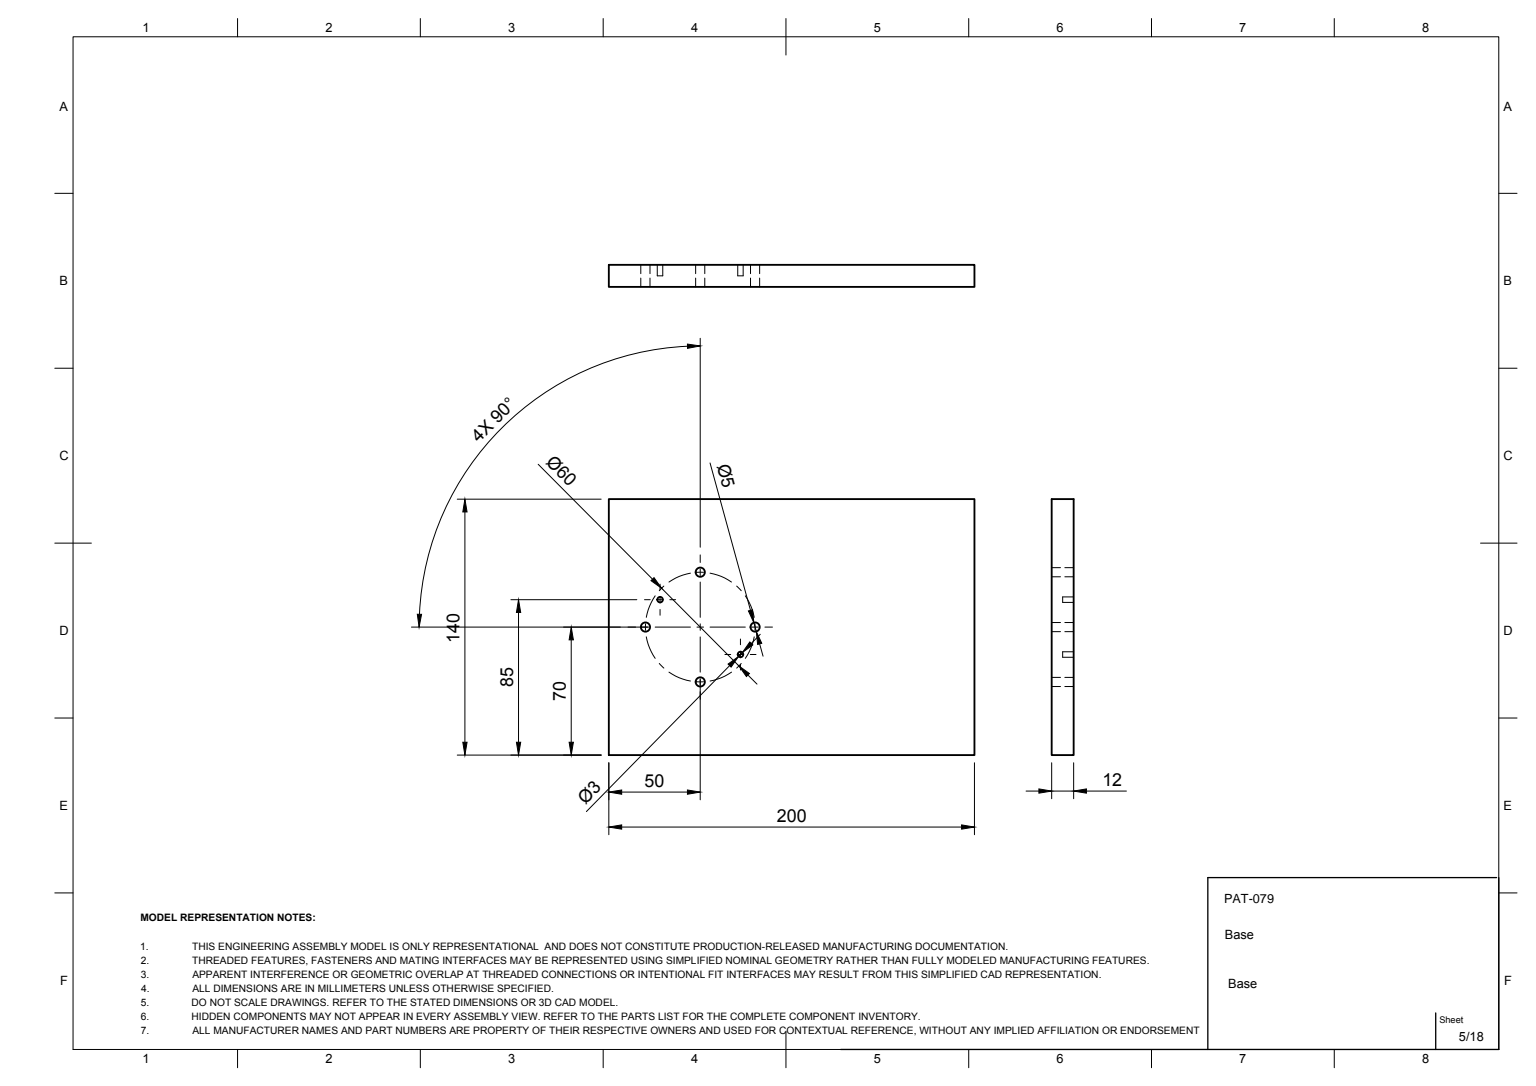
ISO-10303-21;
HEADER;
/* Generated by software containing ST-Developer
 * from STEP Tools, Inc. (www.steptools.com) 
 */

FILE_DESCRIPTION(
/* description */ ('Pipe clamp stand with threaded column'),
/* implementation_level */ '2;1');

FILE_NAME(
/* name */ 'Base.step',
/* time_stamp */ '2026-10-27T10:55:48-07:00',
/* author */ (''),
/* organization */ (''),
/* preprocessor_version */ 'ST-DEVELOPER v20.2',
/* originating_system */ 'Autodesk Translation Framework v15.17.0.0',
/* authorisation */ '');

FILE_SCHEMA (('AUTOMOTIVE_DESIGN { 1 0 10303 214 3 1 1 }'));
ENDSEC;

DATA;
#10=MECHANICAL_DESIGN_GEOMETRIC_PRESENTATION_REPRESENTATION('',(#741),#34433);
#697=SHAPE_REPRESENTATION_RELATIONSHIP('SRR','None',#34539,#719);
#719=ADVANCED_BREP_SHAPE_REPRESENTATION('',(#771),#34407);
#741=STYLED_ITEM('',(#34722),#771);
#771=MANIFOLD_SOLID_BREP('Body1',#8768);
#799=FACE_BOUND('',#1544,.T.);
#800=FACE_BOUND('',#1545,.T.);
#801=FACE_BOUND('',#1546,.T.);
#802=FACE_BOUND('',#1547,.T.);
#803=FACE_BOUND('',#1548,.T.);
#804=FACE_BOUND('',#1549,.T.);
#805=FACE_BOUND('',#1551,.T.);
#806=FACE_BOUND('',#1552,.T.);
#807=FACE_BOUND('',#1553,.T.);
#808=FACE_BOUND('',#1554,.T.);
#857=PLANE('',#9049);
#858=PLANE('',#9053);
#859=PLANE('',#9066);
#860=PLANE('',#9067);
#861=PLANE('',#9068);
#862=PLANE('',#9069);
#863=PLANE('',#9070);
#864=PLANE('',#9071);
#1044=FACE_OUTER_BOUND('',#1531,.T.);
#1045=FACE_OUTER_BOUND('',#1532,.T.);
#1046=FACE_OUTER_BOUND('',#1533,.T.);
#1047=FACE_OUTER_BOUND('',#1534,.T.);
#1048=FACE_OUTER_BOUND('',#1535,.T.);
#1049=FACE_OUTER_BOUND('',#1536,.T.);
#1050=FACE_OUTER_BOUND('',#1537,.T.);
#1051=FACE_OUTER_BOUND('',#1538,.T.);
#1052=FACE_OUTER_BOUND('',#1539,.T.);
#1053=FACE_OUTER_BOUND('',#1540,.T.);
#1054=FACE_OUTER_BOUND('',#1541,.T.);
#1055=FACE_OUTER_BOUND('',#1542,.T.);
#1056=FACE_OUTER_BOUND('',#1543,.T.);
#1057=FACE_OUTER_BOUND('',#1550,.T.);
#1531=EDGE_LOOP('',(#5513,#5514,#5515,#5516));
#1532=EDGE_LOOP('',(#5517));
#1533=EDGE_LOOP('',(#5518,#5519,#5520,#5521));
#1534=EDGE_LOOP('',(#5522));
#1535=EDGE_LOOP('',(#5523,#5524,#5525,#5526));
#1536=EDGE_LOOP('',(#5527,#5528,#5529,#5530));
#1537=EDGE_LOOP('',(#5531,#5532,#5533,#5534));
#1538=EDGE_LOOP('',(#5535,#5536,#5537,#5538));
#1539=EDGE_LOOP('',(#5539,#5540,#5541,#5542));
#1540=EDGE_LOOP('',(#5543,#5544,#5545,#5546));
#1541=EDGE_LOOP('',(#5547,#5548,#5549,#5550));
#1542=EDGE_LOOP('',(#5551,#5552,#5553,#5554));
#1543=EDGE_LOOP('',(#5555,#5556,#5557,#5558));
#1544=EDGE_LOOP('',(#5559));
#1545=EDGE_LOOP('',(#5560));
#1546=EDGE_LOOP('',(#5561));
#1547=EDGE_LOOP('',(#5562));
#1548=EDGE_LOOP('',(#5563));
#1549=EDGE_LOOP('',(#5564));
#1550=EDGE_LOOP('',(#5565,#5566,#5567,#5568));
#1551=EDGE_LOOP('',(#5569));
#1552=EDGE_LOOP('',(#5570));
#1553=EDGE_LOOP('',(#5571));
#1554=EDGE_LOOP('',(#5572));
#2076=LINE('',#11713,#2693);
#2077=LINE('',#11720,#2694);
#2078=LINE('',#11727,#2695);
#2079=LINE('',#11733,#2696);
#2080=LINE('',#11739,#2697);
#2081=LINE('',#11745,#2698);
#2082=LINE('',#11750,#2699);
#2083=LINE('',#11752,#2700);
#2084=LINE('',#11754,#2701);
#2085=LINE('',#11755,#2702);
#2086=LINE('',#11758,#2703);
#2087=LINE('',#11760,#2704);
#2088=LINE('',#11761,#2705);
#2089=LINE('',#11764,#2706);
#2090=LINE('',#11766,#2707);
#2091=LINE('',#11767,#2708);
#2092=LINE('',#11769,#2709);
#2093=LINE('',#11770,#2710);
#2693=VECTOR('',#9735,0.15);
#2694=VECTOR('',#9744,0.15);
#2695=VECTOR('',#9753,0.25);
#2696=VECTOR('',#9760,0.25);
#2697=VECTOR('',#9767,0.25);
#2698=VECTOR('',#9774,0.25);
#2699=VECTOR('',#9779,1.);
#2700=VECTOR('',#9780,1.);
#2701=VECTOR('',#9781,1.);
#2702=VECTOR('',#9782,1.);
#2703=VECTOR('',#9785,1.);
#2704=VECTOR('',#9786,1.);
#2705=VECTOR('',#9787,1.);
#2706=VECTOR('',#9790,1.);
#2707=VECTOR('',#9791,1.);
#2708=VECTOR('',#9792,1.);
#2709=VECTOR('',#9795,1.);
#2710=VECTOR('',#9796,1.);
#3310=CIRCLE('',#9047,0.15);
#3311=CIRCLE('',#9048,0.15);
#3312=CIRCLE('',#9051,0.15);
#3313=CIRCLE('',#9052,0.15);
#3314=CIRCLE('',#9055,0.25);
#3315=CIRCLE('',#9056,0.25);
#3316=CIRCLE('',#9058,0.25);
#3317=CIRCLE('',#9059,0.25);
#3318=CIRCLE('',#9061,0.25);
#3319=CIRCLE('',#9062,0.25);
#3320=CIRCLE('',#9064,0.25);
#3321=CIRCLE('',#9065,0.25);
#3444=VERTEX_POINT('',#11710);
#3445=VERTEX_POINT('',#11712);
#3446=VERTEX_POINT('',#11717);
#3447=VERTEX_POINT('',#11719);
#3448=VERTEX_POINT('',#11724);
#3449=VERTEX_POINT('',#11726);
#3450=VERTEX_POINT('',#11730);
#3451=VERTEX_POINT('',#11732);
#3452=VERTEX_POINT('',#11736);
#3453=VERTEX_POINT('',#11738);
#3454=VERTEX_POINT('',#11742);
#3455=VERTEX_POINT('',#11744);
#3456=VERTEX_POINT('',#11748);
#3457=VERTEX_POINT('',#11749);
#3458=VERTEX_POINT('',#11751);
#3459=VERTEX_POINT('',#11753);
#3460=VERTEX_POINT('',#11757);
#3461=VERTEX_POINT('',#11759);
#3462=VERTEX_POINT('',#11763);
#3463=VERTEX_POINT('',#11765);
#4270=EDGE_CURVE('',#3444,#3444,#3310,.T.);
#4271=EDGE_CURVE('',#3444,#3445,#2076,.T.);
#4272=EDGE_CURVE('',#3445,#3445,#3311,.T.);
#4273=EDGE_CURVE('',#3446,#3446,#3312,.T.);
#4274=EDGE_CURVE('',#3446,#3447,#2077,.T.);
#4275=EDGE_CURVE('',#3447,#3447,#3313,.T.);
#4276=EDGE_CURVE('',#3448,#3448,#3314,.T.);
#4277=EDGE_CURVE('',#3448,#3449,#2078,.T.);
#4278=EDGE_CURVE('',#3449,#3449,#3315,.T.);
#4279=EDGE_CURVE('',#3450,#3450,#3316,.T.);
#4280=EDGE_CURVE('',#3450,#3451,#2079,.T.);
#4281=EDGE_CURVE('',#3451,#3451,#3317,.T.);
#4282=EDGE_CURVE('',#3452,#3452,#3318,.T.);
#4283=EDGE_CURVE('',#3452,#3453,#2080,.T.);
#4284=EDGE_CURVE('',#3453,#3453,#3319,.T.);
#4285=EDGE_CURVE('',#3454,#3454,#3320,.T.);
#4286=EDGE_CURVE('',#3454,#3455,#2081,.T.);
#4287=EDGE_CURVE('',#3455,#3455,#3321,.T.);
#4288=EDGE_CURVE('',#3456,#3457,#2082,.T.);
#4289=EDGE_CURVE('',#3457,#3458,#2083,.T.);
#4290=EDGE_CURVE('',#3459,#3458,#2084,.T.);
#4291=EDGE_CURVE('',#3456,#3459,#2085,.T.);
#4292=EDGE_CURVE('',#3460,#3456,#2086,.T.);
#4293=EDGE_CURVE('',#3461,#3459,#2087,.T.);
#4294=EDGE_CURVE('',#3460,#3461,#2088,.T.);
#4295=EDGE_CURVE('',#3462,#3460,#2089,.T.);
#4296=EDGE_CURVE('',#3463,#3461,#2090,.T.);
#4297=EDGE_CURVE('',#3462,#3463,#2091,.T.);
#4298=EDGE_CURVE('',#3457,#3462,#2092,.T.);
#4299=EDGE_CURVE('',#3458,#3463,#2093,.T.);
#5513=ORIENTED_EDGE('',*,*,#4270,.F.);
#5514=ORIENTED_EDGE('',*,*,#4271,.T.);
#5515=ORIENTED_EDGE('',*,*,#4272,.F.);
#5516=ORIENTED_EDGE('',*,*,#4271,.F.);
#5517=ORIENTED_EDGE('',*,*,#4270,.T.);
#5518=ORIENTED_EDGE('',*,*,#4273,.F.);
#5519=ORIENTED_EDGE('',*,*,#4274,.T.);
#5520=ORIENTED_EDGE('',*,*,#4275,.F.);
#5521=ORIENTED_EDGE('',*,*,#4274,.F.);
#5522=ORIENTED_EDGE('',*,*,#4273,.T.);
#5523=ORIENTED_EDGE('',*,*,#4276,.F.);
#5524=ORIENTED_EDGE('',*,*,#4277,.T.);
#5525=ORIENTED_EDGE('',*,*,#4278,.F.);
#5526=ORIENTED_EDGE('',*,*,#4277,.F.);
#5527=ORIENTED_EDGE('',*,*,#4279,.F.);
#5528=ORIENTED_EDGE('',*,*,#4280,.T.);
#5529=ORIENTED_EDGE('',*,*,#4281,.F.);
#5530=ORIENTED_EDGE('',*,*,#4280,.F.);
#5531=ORIENTED_EDGE('',*,*,#4282,.F.);
#5532=ORIENTED_EDGE('',*,*,#4283,.T.);
#5533=ORIENTED_EDGE('',*,*,#4284,.F.);
#5534=ORIENTED_EDGE('',*,*,#4283,.F.);
#5535=ORIENTED_EDGE('',*,*,#4285,.F.);
#5536=ORIENTED_EDGE('',*,*,#4286,.T.);
#5537=ORIENTED_EDGE('',*,*,#4287,.F.);
#5538=ORIENTED_EDGE('',*,*,#4286,.F.);
#5539=ORIENTED_EDGE('',*,*,#4288,.T.);
#5540=ORIENTED_EDGE('',*,*,#4289,.T.);
#5541=ORIENTED_EDGE('',*,*,#4290,.F.);
#5542=ORIENTED_EDGE('',*,*,#4291,.F.);
#5543=ORIENTED_EDGE('',*,*,#4292,.T.);
#5544=ORIENTED_EDGE('',*,*,#4291,.T.);
#5545=ORIENTED_EDGE('',*,*,#4293,.F.);
#5546=ORIENTED_EDGE('',*,*,#4294,.F.);
#5547=ORIENTED_EDGE('',*,*,#4295,.T.);
#5548=ORIENTED_EDGE('',*,*,#4294,.T.);
#5549=ORIENTED_EDGE('',*,*,#4296,.F.);
#5550=ORIENTED_EDGE('',*,*,#4297,.F.);
#5551=ORIENTED_EDGE('',*,*,#4298,.T.);
#5552=ORIENTED_EDGE('',*,*,#4297,.T.);
#5553=ORIENTED_EDGE('',*,*,#4299,.F.);
#5554=ORIENTED_EDGE('',*,*,#4289,.F.);
#5555=ORIENTED_EDGE('',*,*,#4299,.T.);
#5556=ORIENTED_EDGE('',*,*,#4296,.T.);
#5557=ORIENTED_EDGE('',*,*,#4293,.T.);
#5558=ORIENTED_EDGE('',*,*,#4290,.T.);
#5559=ORIENTED_EDGE('',*,*,#4272,.T.);
#5560=ORIENTED_EDGE('',*,*,#4275,.T.);
#5561=ORIENTED_EDGE('',*,*,#4278,.T.);
#5562=ORIENTED_EDGE('',*,*,#4281,.T.);
#5563=ORIENTED_EDGE('',*,*,#4284,.T.);
#5564=ORIENTED_EDGE('',*,*,#4287,.T.);
#5565=ORIENTED_EDGE('',*,*,#4298,.F.);
#5566=ORIENTED_EDGE('',*,*,#4288,.F.);
#5567=ORIENTED_EDGE('',*,*,#4292,.F.);
#5568=ORIENTED_EDGE('',*,*,#4295,.F.);
#5569=ORIENTED_EDGE('',*,*,#4276,.T.);
#5570=ORIENTED_EDGE('',*,*,#4279,.T.);
#5571=ORIENTED_EDGE('',*,*,#4282,.T.);
#5572=ORIENTED_EDGE('',*,*,#4285,.T.);
#7999=CYLINDRICAL_SURFACE('',#9046,0.15);
#8000=CYLINDRICAL_SURFACE('',#9050,0.15);
#8001=CYLINDRICAL_SURFACE('',#9054,0.25);
#8002=CYLINDRICAL_SURFACE('',#9057,0.25);
#8003=CYLINDRICAL_SURFACE('',#9060,0.25);
#8004=CYLINDRICAL_SURFACE('',#9063,0.25);
#8281=ADVANCED_FACE('',(#1044),#7999,.F.);
#8282=ADVANCED_FACE('',(#1045),#857,.T.);
#8283=ADVANCED_FACE('',(#1046),#8000,.F.);
#8284=ADVANCED_FACE('',(#1047),#858,.T.);
#8285=ADVANCED_FACE('',(#1048),#8001,.F.);
#8286=ADVANCED_FACE('',(#1049),#8002,.F.);
#8287=ADVANCED_FACE('',(#1050),#8003,.F.);
#8288=ADVANCED_FACE('',(#1051),#8004,.F.);
#8289=ADVANCED_FACE('',(#1052),#859,.T.);
#8290=ADVANCED_FACE('',(#1053),#860,.T.);
#8291=ADVANCED_FACE('',(#1054),#861,.T.);
#8292=ADVANCED_FACE('',(#1055),#862,.T.);
#8293=ADVANCED_FACE('',(#1056,#799,#800,#801,#802,#803,#804),#863,.T.);
#8294=ADVANCED_FACE('',(#1057,#805,#806,#807,#808),#864,.F.);
#8768=CLOSED_SHELL('',(#8281,#8282,#8283,#8284,#8285,#8286,#8287,#8288,
#8289,#8290,#8291,#8292,#8293,#8294));
#9045=AXIS2_PLACEMENT_3D('',#11708,#9729,#9730);
#9046=AXIS2_PLACEMENT_3D('',#11709,#9731,#9732);
#9047=AXIS2_PLACEMENT_3D('',#11711,#9733,#9734);
#9048=AXIS2_PLACEMENT_3D('',#11714,#9736,#9737);
#9049=AXIS2_PLACEMENT_3D('',#11715,#9738,#9739);
#9050=AXIS2_PLACEMENT_3D('',#11716,#9740,#9741);
#9051=AXIS2_PLACEMENT_3D('',#11718,#9742,#9743);
#9052=AXIS2_PLACEMENT_3D('',#11721,#9745,#9746);
#9053=AXIS2_PLACEMENT_3D('',#11722,#9747,#9748);
#9054=AXIS2_PLACEMENT_3D('',#11723,#9749,#9750);
#9055=AXIS2_PLACEMENT_3D('',#11725,#9751,#9752);
#9056=AXIS2_PLACEMENT_3D('',#11728,#9754,#9755);
#9057=AXIS2_PLACEMENT_3D('',#11729,#9756,#9757);
#9058=AXIS2_PLACEMENT_3D('',#11731,#9758,#9759);
#9059=AXIS2_PLACEMENT_3D('',#11734,#9761,#9762);
#9060=AXIS2_PLACEMENT_3D('',#11735,#9763,#9764);
#9061=AXIS2_PLACEMENT_3D('',#11737,#9765,#9766);
#9062=AXIS2_PLACEMENT_3D('',#11740,#9768,#9769);
#9063=AXIS2_PLACEMENT_3D('',#11741,#9770,#9771);
#9064=AXIS2_PLACEMENT_3D('',#11743,#9772,#9773);
#9065=AXIS2_PLACEMENT_3D('',#11746,#9775,#9776);
#9066=AXIS2_PLACEMENT_3D('',#11747,#9777,#9778);
#9067=AXIS2_PLACEMENT_3D('',#11756,#9783,#9784);
#9068=AXIS2_PLACEMENT_3D('',#11762,#9788,#9789);
#9069=AXIS2_PLACEMENT_3D('',#11768,#9793,#9794);
#9070=AXIS2_PLACEMENT_3D('',#11771,#9797,#9798);
#9071=AXIS2_PLACEMENT_3D('',#11772,#9799,#9800);
#9729=DIRECTION('axis',(0.,0.,1.));
#9730=DIRECTION('refdir',(1.,0.,0.));
#9731=DIRECTION('center_axis',(0.,0.,1.));
#9732=DIRECTION('ref_axis',(1.,0.,0.));
#9733=DIRECTION('center_axis',(0.,0.,1.));
#9734=DIRECTION('ref_axis',(1.,0.,0.));
#9735=DIRECTION('',(0.,0.,1.));
#9736=DIRECTION('center_axis',(0.,0.,-1.));
#9737=DIRECTION('ref_axis',(1.,0.,0.));
#9738=DIRECTION('center_axis',(0.,0.,1.));
#9739=DIRECTION('ref_axis',(1.,0.,0.));
#9740=DIRECTION('center_axis',(0.,0.,1.));
#9741=DIRECTION('ref_axis',(1.,0.,0.));
#9742=DIRECTION('center_axis',(0.,0.,1.));
#9743=DIRECTION('ref_axis',(1.,0.,0.));
#9744=DIRECTION('',(0.,0.,1.));
#9745=DIRECTION('center_axis',(0.,0.,-1.));
#9746=DIRECTION('ref_axis',(1.,0.,0.));
#9747=DIRECTION('center_axis',(0.,0.,1.));
#9748=DIRECTION('ref_axis',(1.,0.,0.));
#9749=DIRECTION('center_axis',(0.,0.,1.));
#9750=DIRECTION('ref_axis',(1.,0.,0.));
#9751=DIRECTION('center_axis',(0.,0.,1.));
#9752=DIRECTION('ref_axis',(1.,0.,0.));
#9753=DIRECTION('',(0.,0.,1.));
#9754=DIRECTION('center_axis',(0.,0.,-1.));
#9755=DIRECTION('ref_axis',(1.,0.,0.));
#9756=DIRECTION('center_axis',(0.,0.,1.));
#9757=DIRECTION('ref_axis',(1.,0.,0.));
#9758=DIRECTION('center_axis',(0.,0.,1.));
#9759=DIRECTION('ref_axis',(1.,0.,0.));
#9760=DIRECTION('',(0.,0.,1.));
#9761=DIRECTION('center_axis',(0.,0.,-1.));
#9762=DIRECTION('ref_axis',(1.,0.,0.));
#9763=DIRECTION('center_axis',(0.,0.,1.));
#9764=DIRECTION('ref_axis',(1.,0.,0.));
#9765=DIRECTION('center_axis',(0.,0.,1.));
#9766=DIRECTION('ref_axis',(1.,0.,0.));
#9767=DIRECTION('',(0.,0.,1.));
#9768=DIRECTION('center_axis',(0.,0.,-1.));
#9769=DIRECTION('ref_axis',(1.,0.,0.));
#9770=DIRECTION('center_axis',(0.,0.,1.));
#9771=DIRECTION('ref_axis',(1.,0.,0.));
#9772=DIRECTION('center_axis',(0.,0.,1.));
#9773=DIRECTION('ref_axis',(1.,0.,0.));
#9774=DIRECTION('',(0.,0.,1.));
#9775=DIRECTION('center_axis',(0.,0.,-1.));
#9776=DIRECTION('ref_axis',(1.,0.,0.));
#9777=DIRECTION('center_axis',(0.,1.,0.));
#9778=DIRECTION('ref_axis',(-1.,0.,0.));
#9779=DIRECTION('',(-1.,0.,0.));
#9780=DIRECTION('',(0.,0.,1.));
#9781=DIRECTION('',(-1.,0.,0.));
#9782=DIRECTION('',(0.,0.,1.));
#9783=DIRECTION('center_axis',(1.,0.,0.));
#9784=DIRECTION('ref_axis',(0.,1.,0.));
#9785=DIRECTION('',(0.,1.,0.));
#9786=DIRECTION('',(0.,1.,0.));
#9787=DIRECTION('',(0.,0.,1.));
#9788=DIRECTION('center_axis',(0.,-1.,0.));
#9789=DIRECTION('ref_axis',(1.,0.,0.));
#9790=DIRECTION('',(1.,0.,0.));
#9791=DIRECTION('',(1.,0.,0.));
#9792=DIRECTION('',(0.,0.,1.));
#9793=DIRECTION('center_axis',(-1.,0.,0.));
#9794=DIRECTION('ref_axis',(0.,-1.,0.));
#9795=DIRECTION('',(0.,-1.,0.));
#9796=DIRECTION('',(0.,-1.,0.));
#9797=DIRECTION('center_axis',(0.,0.,1.));
#9798=DIRECTION('ref_axis',(1.,0.,0.));
#9799=DIRECTION('center_axis',(0.,0.,1.));
#9800=DIRECTION('ref_axis',(1.,0.,0.));
#11708=CARTESIAN_POINT('',(0.,0.,0.));
#11709=CARTESIAN_POINT('Origin',(-6.3,-1.5,0.6));
#11710=CARTESIAN_POINT('',(-6.45,-1.5,0.6));
#11711=CARTESIAN_POINT('Origin',(-6.3,-1.5,0.6));
#11712=CARTESIAN_POINT('',(-6.45,-1.5,1.2));
#11713=CARTESIAN_POINT('',(-6.45,-1.5,0.6));
#11714=CARTESIAN_POINT('Origin',(-6.3,-1.5,1.2));
#11715=CARTESIAN_POINT('Origin',(-6.3,-1.5,0.6));
#11716=CARTESIAN_POINT('Origin',(-10.7,1.5,0.6));
#11717=CARTESIAN_POINT('',(-10.85,1.5,0.6));
#11718=CARTESIAN_POINT('Origin',(-10.7,1.5,0.6));
#11719=CARTESIAN_POINT('',(-10.85,1.5,1.2));
#11720=CARTESIAN_POINT('',(-10.85,1.5,0.6));
#11721=CARTESIAN_POINT('Origin',(-10.7,1.5,1.2));
#11722=CARTESIAN_POINT('Origin',(-10.7,1.5,0.6));
#11723=CARTESIAN_POINT('Origin',(-11.5,3.67394039744206E-16,-0.1));
#11724=CARTESIAN_POINT('',(-11.75,3.36777869765522E-16,0.));
#11725=CARTESIAN_POINT('Origin',(-11.5,3.67394039744206E-16,0.));
#11726=CARTESIAN_POINT('',(-11.75,3.9801020972289E-16,1.2));
#11727=CARTESIAN_POINT('',(-11.75,3.36777869765522E-16,-0.1));
#11728=CARTESIAN_POINT('Origin',(-11.5,3.67394039744206E-16,1.2));
#11729=CARTESIAN_POINT('Origin',(-8.5,3.,-0.1));
#11730=CARTESIAN_POINT('',(-8.75,3.,0.));
#11731=CARTESIAN_POINT('Origin',(-8.5,3.,0.));
#11732=CARTESIAN_POINT('',(-8.75,3.,1.2));
#11733=CARTESIAN_POINT('',(-8.75,3.,-0.1));
#11734=CARTESIAN_POINT('Origin',(-8.5,3.,1.2));
#11735=CARTESIAN_POINT('Origin',(-5.5,0.,-0.1));
#11736=CARTESIAN_POINT('',(-5.75,-3.06161699786838E-17,0.));
#11737=CARTESIAN_POINT('Origin',(-5.5,0.,0.));
#11738=CARTESIAN_POINT('',(-5.75,3.06161699786838E-17,1.2));
#11739=CARTESIAN_POINT('',(-5.75,-3.06161699786838E-17,-0.1));
#11740=CARTESIAN_POINT('Origin',(-5.5,0.,1.2));
#11741=CARTESIAN_POINT('Origin',(-8.5,-3.,-0.1));
#11742=CARTESIAN_POINT('',(-8.75,-3.,0.));
#11743=CARTESIAN_POINT('Origin',(-8.5,-3.,0.));
#11744=CARTESIAN_POINT('',(-8.75,-3.,1.2));
#11745=CARTESIAN_POINT('',(-8.75,-3.,-0.1));
#11746=CARTESIAN_POINT('Origin',(-8.5,-3.,1.2));
#11747=CARTESIAN_POINT('Origin',(6.5,7.,0.));
#11748=CARTESIAN_POINT('',(6.5,7.,0.));
#11749=CARTESIAN_POINT('',(-13.5,7.,0.));
#11750=CARTESIAN_POINT('',(6.5,7.,0.));
#11751=CARTESIAN_POINT('',(-13.5,7.,1.2));
#11752=CARTESIAN_POINT('',(-13.5,7.,0.));
#11753=CARTESIAN_POINT('',(6.5,7.,1.2));
#11754=CARTESIAN_POINT('',(6.5,7.,1.2));
#11755=CARTESIAN_POINT('',(6.5,7.,0.));
#11756=CARTESIAN_POINT('Origin',(6.5,-7.,0.));
#11757=CARTESIAN_POINT('',(6.5,-7.,0.));
#11758=CARTESIAN_POINT('',(6.5,-7.,0.));
#11759=CARTESIAN_POINT('',(6.5,-7.,1.2));
#11760=CARTESIAN_POINT('',(6.5,-7.,1.2));
#11761=CARTESIAN_POINT('',(6.5,-7.,0.));
#11762=CARTESIAN_POINT('Origin',(-13.5,-7.,0.));
#11763=CARTESIAN_POINT('',(-13.5,-7.,0.));
#11764=CARTESIAN_POINT('',(-13.5,-7.,0.));
#11765=CARTESIAN_POINT('',(-13.5,-7.,1.2));
#11766=CARTESIAN_POINT('',(-13.5,-7.,1.2));
#11767=CARTESIAN_POINT('',(-13.5,-7.,0.));
#11768=CARTESIAN_POINT('Origin',(-13.5,7.,0.));
#11769=CARTESIAN_POINT('',(-13.5,7.,0.));
#11770=CARTESIAN_POINT('',(-13.5,7.,1.2));
#11771=CARTESIAN_POINT('Origin',(-3.5,0.,1.2));
#11772=CARTESIAN_POINT('Origin',(-3.5,0.,0.));
#34378=UNCERTAINTY_MEASURE_WITH_UNIT(LENGTH_MEASURE(0.001),#34434,
'DISTANCE_ACCURACY_VALUE',
'Maximum model space distance between geometric entities at asserted c
onnectivities');
#34404=UNCERTAINTY_MEASURE_WITH_UNIT(LENGTH_MEASURE(0.001),#34434,
'DISTANCE_ACCURACY_VALUE',
'Maximum model space distance between geometric entities at asserted c
onnectivities');
#34407=(
GEOMETRIC_REPRESENTATION_CONTEXT(3)
GLOBAL_UNCERTAINTY_ASSIGNED_CONTEXT((#34378))
GLOBAL_UNIT_ASSIGNED_CONTEXT((#34434,#34436,#34437))
REPRESENTATION_CONTEXT('','3D')
);
#34433=(
GEOMETRIC_REPRESENTATION_CONTEXT(3)
GLOBAL_UNCERTAINTY_ASSIGNED_CONTEXT((#34404))
GLOBAL_UNIT_ASSIGNED_CONTEXT((#34434,#34436,#34437))
REPRESENTATION_CONTEXT('','3D')
);
#34434=(
LENGTH_UNIT()
NAMED_UNIT(*)
SI_UNIT(.CENTI.,.METRE.)
);
#34436=(
NAMED_UNIT(*)
PLANE_ANGLE_UNIT()
SI_UNIT($,.RADIAN.)
);
#34437=(
NAMED_UNIT(*)
SI_UNIT($,.STERADIAN.)
SOLID_ANGLE_UNIT()
);
#34440=SHAPE_DEFINITION_REPRESENTATION(#34468,#34539);
#34468=PRODUCT_DEFINITION_SHAPE('',$,#34568);
#34539=SHAPE_REPRESENTATION('',(#9045),#34407);
#34565=PRODUCT_DEFINITION_CONTEXT('part definition',#34651,'design');
#34568=PRODUCT_DEFINITION('Base','Base',#34596,#34565);
#34596=PRODUCT_DEFINITION_FORMATION('',$,#34655);
#34651=APPLICATION_CONTEXT(
'Core Data for Automotive Mechanical Design Process');
#34652=PRODUCT_CONTEXT('part definition',#34651,'mechanical');
#34655=PRODUCT('Base','Base','Base',(#34652));
#34716=COLOUR_RGB('Dark Blue',0.08,0.2,0.34);
#34717=FILL_AREA_STYLE_COLOUR('',#34716);
#34718=FILL_AREA_STYLE('',(#34717));
#34719=SURFACE_STYLE_FILL_AREA(#34718);
#34720=SURFACE_SIDE_STYLE('',(#34719));
#34721=SURFACE_STYLE_USAGE(.BOTH.,#34720);
#34722=PRESENTATION_STYLE_ASSIGNMENT((#34721));
ENDSEC;
END-ISO-10303-21;
